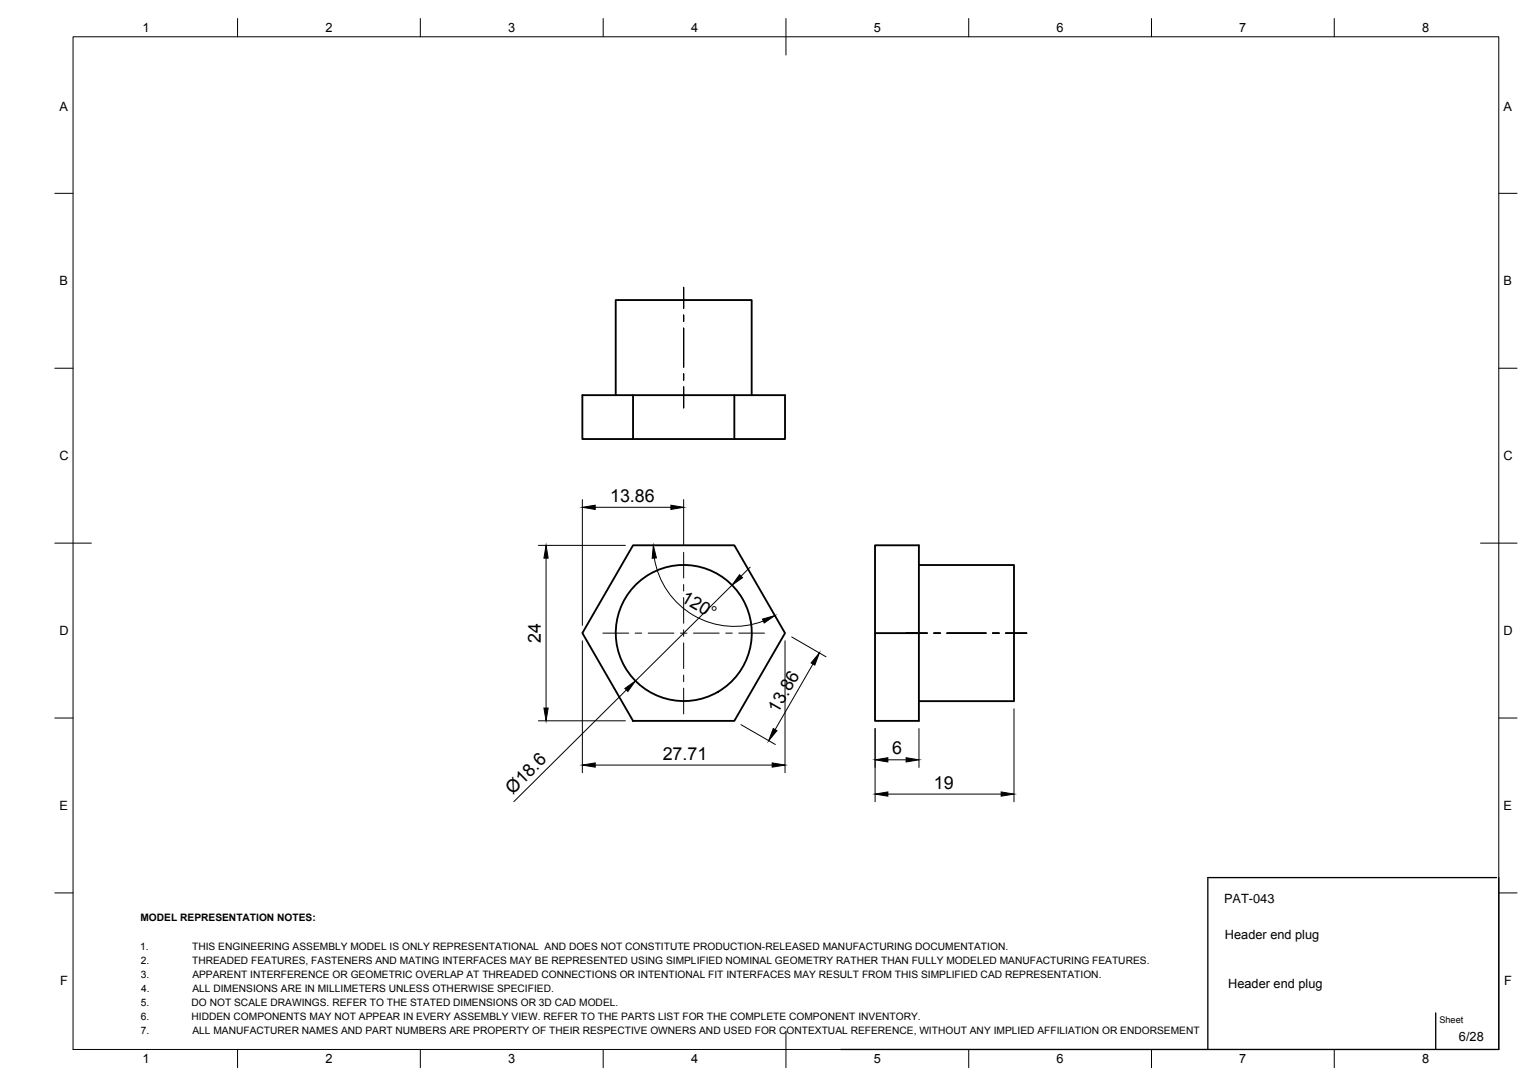
ISO-10303-21;
HEADER;
/* Generated by software containing ST-Developer
 * from STEP Tools, Inc. (www.steptools.com) 
 */

FILE_DESCRIPTION(
/* description */ ('Four-valve pipe header'),
/* implementation_level */ '2;1');

FILE_NAME(
/* name */ 'Header end plug.step',
/* time_stamp */ '2026-10-29T16:56:19-07:00',
/* author */ (''),
/* organization */ (''),
/* preprocessor_version */ 'ST-DEVELOPER v20.2',
/* originating_system */ 'Autodesk Translation Framework v15.17.0.0',
/* authorisation */ '');

FILE_SCHEMA (('AUTOMOTIVE_DESIGN { 1 0 10303 214 3 1 1 }'));
ENDSEC;

DATA;
#10=MECHANICAL_DESIGN_GEOMETRIC_PRESENTATION_REPRESENTATION('',(#334),#10119);
#282=SHAPE_REPRESENTATION_RELATIONSHIP('SRR','None',#10243,#308);
#308=ADVANCED_BREP_SHAPE_REPRESENTATION('',(#360),#10092);
#334=STYLED_ITEM('',(#10484),#360);
#360=MANIFOLD_SOLID_BREP('Body1',#5580);
#436=FACE_BOUND('',#1141,.T.);
#561=PLANE('',#6020);
#562=PLANE('',#6022);
#563=PLANE('',#6023);
#564=PLANE('',#6024);
#565=PLANE('',#6025);
#566=PLANE('',#6026);
#567=PLANE('',#6027);
#568=PLANE('',#6028);
#569=PLANE('',#6031);
#798=FACE_OUTER_BOUND('',#1140,.T.);
#799=FACE_OUTER_BOUND('',#1142,.T.);
#800=FACE_OUTER_BOUND('',#1143,.T.);
#801=FACE_OUTER_BOUND('',#1144,.T.);
#802=FACE_OUTER_BOUND('',#1145,.T.);
#803=FACE_OUTER_BOUND('',#1146,.T.);
#804=FACE_OUTER_BOUND('',#1147,.T.);
#805=FACE_OUTER_BOUND('',#1148,.T.);
#806=FACE_OUTER_BOUND('',#1149,.T.);
#807=FACE_OUTER_BOUND('',#1150,.T.);
#1140=EDGE_LOOP('',(#4003,#4004,#4005,#4006,#4007,#4008));
#1141=EDGE_LOOP('',(#4009));
#1142=EDGE_LOOP('',(#4010,#4011,#4012,#4013));
#1143=EDGE_LOOP('',(#4014,#4015,#4016,#4017));
#1144=EDGE_LOOP('',(#4018,#4019,#4020,#4021));
#1145=EDGE_LOOP('',(#4022,#4023,#4024,#4025));
#1146=EDGE_LOOP('',(#4026,#4027,#4028,#4029));
#1147=EDGE_LOOP('',(#4030,#4031,#4032,#4033));
#1148=EDGE_LOOP('',(#4034,#4035,#4036,#4037,#4038,#4039));
#1149=EDGE_LOOP('',(#4040,#4041,#4042,#4043));
#1150=EDGE_LOOP('',(#4044));
#1569=LINE('',#8714,#1987);
#1570=LINE('',#8716,#1988);
#1571=LINE('',#8718,#1989);
#1572=LINE('',#8720,#1990);
#1573=LINE('',#8722,#1991);
#1574=LINE('',#8723,#1992);
#1575=LINE('',#8729,#1993);
#1576=LINE('',#8730,#1994);
#1577=LINE('',#8731,#1995);
#1578=LINE('',#8734,#1996);
#1579=LINE('',#8735,#1997);
#1580=LINE('',#8738,#1998);
#1581=LINE('',#8739,#1999);
#1582=LINE('',#8742,#2000);
#1583=LINE('',#8743,#2001);
#1584=LINE('',#8746,#2002);
#1585=LINE('',#8747,#2003);
#1586=LINE('',#8749,#2004);
#1587=LINE('',#8754,#2005);
#1987=VECTOR('',#6870,1.);
#1988=VECTOR('',#6871,1.);
#1989=VECTOR('',#6872,1.);
#1990=VECTOR('',#6873,1.);
#1991=VECTOR('',#6874,1.);
#1992=VECTOR('',#6875,1.);
#1993=VECTOR('',#6880,1.);
#1994=VECTOR('',#6881,1.);
#1995=VECTOR('',#6882,1.);
#1996=VECTOR('',#6885,1.);
#1997=VECTOR('',#6886,1.);
#1998=VECTOR('',#6889,1.);
#1999=VECTOR('',#6890,1.);
#2000=VECTOR('',#6893,1.);
#2001=VECTOR('',#6894,1.);
#2002=VECTOR('',#6897,1.);
#2003=VECTOR('',#6898,1.);
#2004=VECTOR('',#6901,1.);
#2005=VECTOR('',#6908,0.93);
#2394=CIRCLE('',#6021,0.93);
#2395=CIRCLE('',#6030,0.93);
#2662=VERTEX_POINT('',#8712);
#2663=VERTEX_POINT('',#8713);
#2664=VERTEX_POINT('',#8715);
#2665=VERTEX_POINT('',#8717);
#2666=VERTEX_POINT('',#8719);
#2667=VERTEX_POINT('',#8721);
#2668=VERTEX_POINT('',#8724);
#2669=VERTEX_POINT('',#8727);
#2670=VERTEX_POINT('',#8728);
#2671=VERTEX_POINT('',#8733);
#2672=VERTEX_POINT('',#8737);
#2673=VERTEX_POINT('',#8741);
#2674=VERTEX_POINT('',#8745);
#2675=VERTEX_POINT('',#8752);
#3168=EDGE_CURVE('',#2662,#2663,#1569,.T.);
#3169=EDGE_CURVE('',#2663,#2664,#1570,.T.);
#3170=EDGE_CURVE('',#2664,#2665,#1571,.T.);
#3171=EDGE_CURVE('',#2665,#2666,#1572,.T.);
#3172=EDGE_CURVE('',#2666,#2667,#1573,.T.);
#3173=EDGE_CURVE('',#2667,#2662,#1574,.T.);
#3174=EDGE_CURVE('',#2668,#2668,#2394,.T.);
#3175=EDGE_CURVE('',#2669,#2670,#1575,.T.);
#3176=EDGE_CURVE('',#2670,#2662,#1576,.T.);
#3177=EDGE_CURVE('',#2669,#2667,#1577,.T.);
#3178=EDGE_CURVE('',#2671,#2669,#1578,.T.);
#3179=EDGE_CURVE('',#2671,#2666,#1579,.T.);
#3180=EDGE_CURVE('',#2672,#2671,#1580,.T.);
#3181=EDGE_CURVE('',#2672,#2665,#1581,.T.);
#3182=EDGE_CURVE('',#2673,#2672,#1582,.T.);
#3183=EDGE_CURVE('',#2673,#2664,#1583,.T.);
#3184=EDGE_CURVE('',#2674,#2673,#1584,.T.);
#3185=EDGE_CURVE('',#2674,#2663,#1585,.T.);
#3186=EDGE_CURVE('',#2670,#2674,#1586,.T.);
#3187=EDGE_CURVE('',#2675,#2675,#2395,.T.);
#3188=EDGE_CURVE('',#2675,#2668,#1587,.T.);
#4003=ORIENTED_EDGE('',*,*,#3168,.T.);
#4004=ORIENTED_EDGE('',*,*,#3169,.T.);
#4005=ORIENTED_EDGE('',*,*,#3170,.T.);
#4006=ORIENTED_EDGE('',*,*,#3171,.T.);
#4007=ORIENTED_EDGE('',*,*,#3172,.T.);
#4008=ORIENTED_EDGE('',*,*,#3173,.T.);
#4009=ORIENTED_EDGE('',*,*,#3174,.F.);
#4010=ORIENTED_EDGE('',*,*,#3175,.T.);
#4011=ORIENTED_EDGE('',*,*,#3176,.T.);
#4012=ORIENTED_EDGE('',*,*,#3173,.F.);
#4013=ORIENTED_EDGE('',*,*,#3177,.F.);
#4014=ORIENTED_EDGE('',*,*,#3178,.T.);
#4015=ORIENTED_EDGE('',*,*,#3177,.T.);
#4016=ORIENTED_EDGE('',*,*,#3172,.F.);
#4017=ORIENTED_EDGE('',*,*,#3179,.F.);
#4018=ORIENTED_EDGE('',*,*,#3180,.T.);
#4019=ORIENTED_EDGE('',*,*,#3179,.T.);
#4020=ORIENTED_EDGE('',*,*,#3171,.F.);
#4021=ORIENTED_EDGE('',*,*,#3181,.F.);
#4022=ORIENTED_EDGE('',*,*,#3182,.T.);
#4023=ORIENTED_EDGE('',*,*,#3181,.T.);
#4024=ORIENTED_EDGE('',*,*,#3170,.F.);
#4025=ORIENTED_EDGE('',*,*,#3183,.F.);
#4026=ORIENTED_EDGE('',*,*,#3184,.T.);
#4027=ORIENTED_EDGE('',*,*,#3183,.T.);
#4028=ORIENTED_EDGE('',*,*,#3169,.F.);
#4029=ORIENTED_EDGE('',*,*,#3185,.F.);
#4030=ORIENTED_EDGE('',*,*,#3186,.T.);
#4031=ORIENTED_EDGE('',*,*,#3185,.T.);
#4032=ORIENTED_EDGE('',*,*,#3168,.F.);
#4033=ORIENTED_EDGE('',*,*,#3176,.F.);
#4034=ORIENTED_EDGE('',*,*,#3186,.F.);
#4035=ORIENTED_EDGE('',*,*,#3175,.F.);
#4036=ORIENTED_EDGE('',*,*,#3178,.F.);
#4037=ORIENTED_EDGE('',*,*,#3180,.F.);
#4038=ORIENTED_EDGE('',*,*,#3182,.F.);
#4039=ORIENTED_EDGE('',*,*,#3184,.F.);
#4040=ORIENTED_EDGE('',*,*,#3187,.F.);
#4041=ORIENTED_EDGE('',*,*,#3188,.T.);
#4042=ORIENTED_EDGE('',*,*,#3174,.T.);
#4043=ORIENTED_EDGE('',*,*,#3188,.F.);
#4044=ORIENTED_EDGE('',*,*,#3187,.T.);
#5174=CYLINDRICAL_SURFACE('',#6029,0.93);
#5298=ADVANCED_FACE('',(#798,#436),#561,.T.);
#5299=ADVANCED_FACE('',(#799),#562,.T.);
#5300=ADVANCED_FACE('',(#800),#563,.T.);
#5301=ADVANCED_FACE('',(#801),#564,.T.);
#5302=ADVANCED_FACE('',(#802),#565,.T.);
#5303=ADVANCED_FACE('',(#803),#566,.T.);
#5304=ADVANCED_FACE('',(#804),#567,.T.);
#5305=ADVANCED_FACE('',(#805),#568,.F.);
#5306=ADVANCED_FACE('',(#806),#5174,.T.);
#5307=ADVANCED_FACE('',(#807),#569,.T.);
#5580=CLOSED_SHELL('',(#5298,#5299,#5300,#5301,#5302,#5303,#5304,#5305,
#5306,#5307));
#6019=AXIS2_PLACEMENT_3D('',#8710,#6866,#6867);
#6020=AXIS2_PLACEMENT_3D('',#8711,#6868,#6869);
#6021=AXIS2_PLACEMENT_3D('',#8725,#6876,#6877);
#6022=AXIS2_PLACEMENT_3D('',#8726,#6878,#6879);
#6023=AXIS2_PLACEMENT_3D('',#8732,#6883,#6884);
#6024=AXIS2_PLACEMENT_3D('',#8736,#6887,#6888);
#6025=AXIS2_PLACEMENT_3D('',#8740,#6891,#6892);
#6026=AXIS2_PLACEMENT_3D('',#8744,#6895,#6896);
#6027=AXIS2_PLACEMENT_3D('',#8748,#6899,#6900);
#6028=AXIS2_PLACEMENT_3D('',#8750,#6902,#6903);
#6029=AXIS2_PLACEMENT_3D('',#8751,#6904,#6905);
#6030=AXIS2_PLACEMENT_3D('',#8753,#6906,#6907);
#6031=AXIS2_PLACEMENT_3D('',#8755,#6909,#6910);
#6866=DIRECTION('axis',(0.,0.,1.));
#6867=DIRECTION('refdir',(1.,0.,0.));
#6868=DIRECTION('center_axis',(1.,0.,0.));
#6869=DIRECTION('ref_axis',(0.,0.,-1.));
#6870=DIRECTION('',(0.,0.5,0.866025403784439));
#6871=DIRECTION('',(0.,-0.5,0.866025403784439));
#6872=DIRECTION('',(0.,-1.,0.));
#6873=DIRECTION('',(0.,-0.500000000000001,-0.866025403784438));
#6874=DIRECTION('',(0.,0.5,-0.866025403784439));
#6875=DIRECTION('',(0.,1.,0.));
#6876=DIRECTION('center_axis',(1.,0.,0.));
#6877=DIRECTION('ref_axis',(0.,0.,-1.));
#6878=DIRECTION('center_axis',(0.,0.,-1.));
#6879=DIRECTION('ref_axis',(0.,1.,0.));
#6880=DIRECTION('',(0.,1.,0.));
#6881=DIRECTION('',(1.,0.,0.));
#6882=DIRECTION('',(1.,0.,0.));
#6883=DIRECTION('center_axis',(0.,-0.866025403784439,-0.5));
#6884=DIRECTION('ref_axis',(0.,0.5,-0.866025403784439));
#6885=DIRECTION('',(0.,0.5,-0.866025403784439));
#6886=DIRECTION('',(1.,0.,0.));
#6887=DIRECTION('center_axis',(0.,-0.866025403784438,0.500000000000001));
#6888=DIRECTION('ref_axis',(0.,-0.500000000000001,-0.866025403784438));
#6889=DIRECTION('',(0.,-0.500000000000001,-0.866025403784438));
#6890=DIRECTION('',(1.,0.,0.));
#6891=DIRECTION('center_axis',(0.,0.,1.));
#6892=DIRECTION('ref_axis',(0.,-1.,0.));
#6893=DIRECTION('',(0.,-1.,0.));
#6894=DIRECTION('',(1.,0.,0.));
#6895=DIRECTION('center_axis',(0.,0.866025403784439,0.5));
#6896=DIRECTION('ref_axis',(0.,-0.5,0.866025403784439));
#6897=DIRECTION('',(0.,-0.5,0.866025403784439));
#6898=DIRECTION('',(1.,0.,0.));
#6899=DIRECTION('center_axis',(0.,0.866025403784439,-0.5));
#6900=DIRECTION('ref_axis',(0.,0.5,0.866025403784439));
#6901=DIRECTION('',(0.,0.5,0.866025403784439));
#6902=DIRECTION('center_axis',(1.,0.,0.));
#6903=DIRECTION('ref_axis',(0.,0.,-1.));
#6904=DIRECTION('center_axis',(1.,0.,0.));
#6905=DIRECTION('ref_axis',(0.,0.,-1.));
#6906=DIRECTION('center_axis',(1.,0.,0.));
#6907=DIRECTION('ref_axis',(0.,0.,-1.));
#6908=DIRECTION('',(-1.,0.,0.));
#6909=DIRECTION('center_axis',(1.,0.,0.));
#6910=DIRECTION('ref_axis',(0.,0.,-1.));
#8710=CARTESIAN_POINT('',(0.,0.,0.));
#8711=CARTESIAN_POINT('Origin',(-4.,7.75,5.));
#8712=CARTESIAN_POINT('',(-4.,8.44282032302755,3.8));
#8713=CARTESIAN_POINT('',(-4.,9.1356406460551,5.));
#8714=CARTESIAN_POINT('',(-4.,8.44282032302755,3.8));
#8715=CARTESIAN_POINT('',(-4.,8.44282032302755,6.2));
#8716=CARTESIAN_POINT('',(-4.,9.1356406460551,5.));
#8717=CARTESIAN_POINT('',(-4.,7.05717967697245,6.2));
#8718=CARTESIAN_POINT('',(-4.,8.44282032302755,6.2));
#8719=CARTESIAN_POINT('',(-4.,6.3643593539449,5.));
#8720=CARTESIAN_POINT('',(-4.,7.05717967697245,6.2));
#8721=CARTESIAN_POINT('',(-4.,7.05717967697245,3.8));
#8722=CARTESIAN_POINT('',(-4.,6.3643593539449,5.));
#8723=CARTESIAN_POINT('',(-4.,7.05717967697245,3.8));
#8724=CARTESIAN_POINT('',(-4.,7.75,5.93));
#8725=CARTESIAN_POINT('Origin',(-4.,7.75,5.));
#8726=CARTESIAN_POINT('Origin',(-4.6,7.05717967697245,3.8));
#8727=CARTESIAN_POINT('',(-4.6,7.05717967697245,3.8));
#8728=CARTESIAN_POINT('',(-4.6,8.44282032302755,3.8));
#8729=CARTESIAN_POINT('',(-4.6,7.05717967697245,3.8));
#8730=CARTESIAN_POINT('',(-4.6,8.44282032302755,3.8));
#8731=CARTESIAN_POINT('',(-4.6,7.05717967697245,3.8));
#8732=CARTESIAN_POINT('Origin',(-4.6,6.3643593539449,5.));
#8733=CARTESIAN_POINT('',(-4.6,6.3643593539449,5.));
#8734=CARTESIAN_POINT('',(-4.6,6.3643593539449,5.));
#8735=CARTESIAN_POINT('',(-4.6,6.3643593539449,5.));
#8736=CARTESIAN_POINT('Origin',(-4.6,7.05717967697245,6.2));
#8737=CARTESIAN_POINT('',(-4.6,7.05717967697245,6.2));
#8738=CARTESIAN_POINT('',(-4.6,7.05717967697245,6.2));
#8739=CARTESIAN_POINT('',(-4.6,7.05717967697245,6.2));
#8740=CARTESIAN_POINT('Origin',(-4.6,8.44282032302755,6.2));
#8741=CARTESIAN_POINT('',(-4.6,8.44282032302755,6.2));
#8742=CARTESIAN_POINT('',(-4.6,8.44282032302755,6.2));
#8743=CARTESIAN_POINT('',(-4.6,8.44282032302755,6.2));
#8744=CARTESIAN_POINT('Origin',(-4.6,9.1356406460551,5.));
#8745=CARTESIAN_POINT('',(-4.6,9.1356406460551,5.));
#8746=CARTESIAN_POINT('',(-4.6,9.1356406460551,5.));
#8747=CARTESIAN_POINT('',(-4.6,9.1356406460551,5.));
#8748=CARTESIAN_POINT('Origin',(-4.6,8.44282032302755,3.8));
#8749=CARTESIAN_POINT('',(-4.6,8.44282032302755,3.8));
#8750=CARTESIAN_POINT('Origin',(-4.6,7.75,5.));
#8751=CARTESIAN_POINT('Origin',(-4.,7.75,5.));
#8752=CARTESIAN_POINT('',(-2.7,7.75,5.93));
#8753=CARTESIAN_POINT('Origin',(-2.7,7.75,5.));
#8754=CARTESIAN_POINT('',(-4.,7.75,5.93));
#8755=CARTESIAN_POINT('Origin',(-2.7,7.75,5.));
#10061=UNCERTAINTY_MEASURE_WITH_UNIT(LENGTH_MEASURE(0.001),#10120,
'DISTANCE_ACCURACY_VALUE',
'Maximum model space distance between geometric entities at asserted c
onnectivities');
#10088=UNCERTAINTY_MEASURE_WITH_UNIT(LENGTH_MEASURE(0.001),#10120,
'DISTANCE_ACCURACY_VALUE',
'Maximum model space distance between geometric entities at asserted c
onnectivities');
#10092=(
GEOMETRIC_REPRESENTATION_CONTEXT(3)
GLOBAL_UNCERTAINTY_ASSIGNED_CONTEXT((#10061))
GLOBAL_UNIT_ASSIGNED_CONTEXT((#10120,#10122,#10123))
REPRESENTATION_CONTEXT('','3D')
);
#10119=(
GEOMETRIC_REPRESENTATION_CONTEXT(3)
GLOBAL_UNCERTAINTY_ASSIGNED_CONTEXT((#10088))
GLOBAL_UNIT_ASSIGNED_CONTEXT((#10120,#10122,#10123))
REPRESENTATION_CONTEXT('','3D')
);
#10120=(
LENGTH_UNIT()
NAMED_UNIT(*)
SI_UNIT(.CENTI.,.METRE.)
);
#10122=(
NAMED_UNIT(*)
PLANE_ANGLE_UNIT()
SI_UNIT($,.RADIAN.)
);
#10123=(
NAMED_UNIT(*)
SI_UNIT($,.STERADIAN.)
SOLID_ANGLE_UNIT()
);
#10127=SHAPE_DEFINITION_REPRESENTATION(#10157,#10243);
#10157=PRODUCT_DEFINITION_SHAPE('',$,#10274);
#10243=SHAPE_REPRESENTATION('',(#6019),#10092);
#10270=PRODUCT_DEFINITION_CONTEXT('part definition',#10362,'design');
#10274=PRODUCT_DEFINITION('Header end plug','Header end plug',#10304,#10270);
#10304=PRODUCT_DEFINITION_FORMATION('',$,#10367);
#10362=APPLICATION_CONTEXT(
'Core Data for Automotive Mechanical Design Process');
#10363=PRODUCT_CONTEXT('part definition',#10362,'mechanical');
#10367=PRODUCT('Header end plug','Header end plug','Header end plug',(#10363));
#10478=COLOUR_RGB('Off White',0.89,0.88,0.83);
#10479=FILL_AREA_STYLE_COLOUR('',#10478);
#10480=FILL_AREA_STYLE('',(#10479));
#10481=SURFACE_STYLE_FILL_AREA(#10480);
#10482=SURFACE_SIDE_STYLE('',(#10481));
#10483=SURFACE_STYLE_USAGE(.BOTH.,#10482);
#10484=PRESENTATION_STYLE_ASSIGNMENT((#10483));
ENDSEC;
END-ISO-10303-21;
